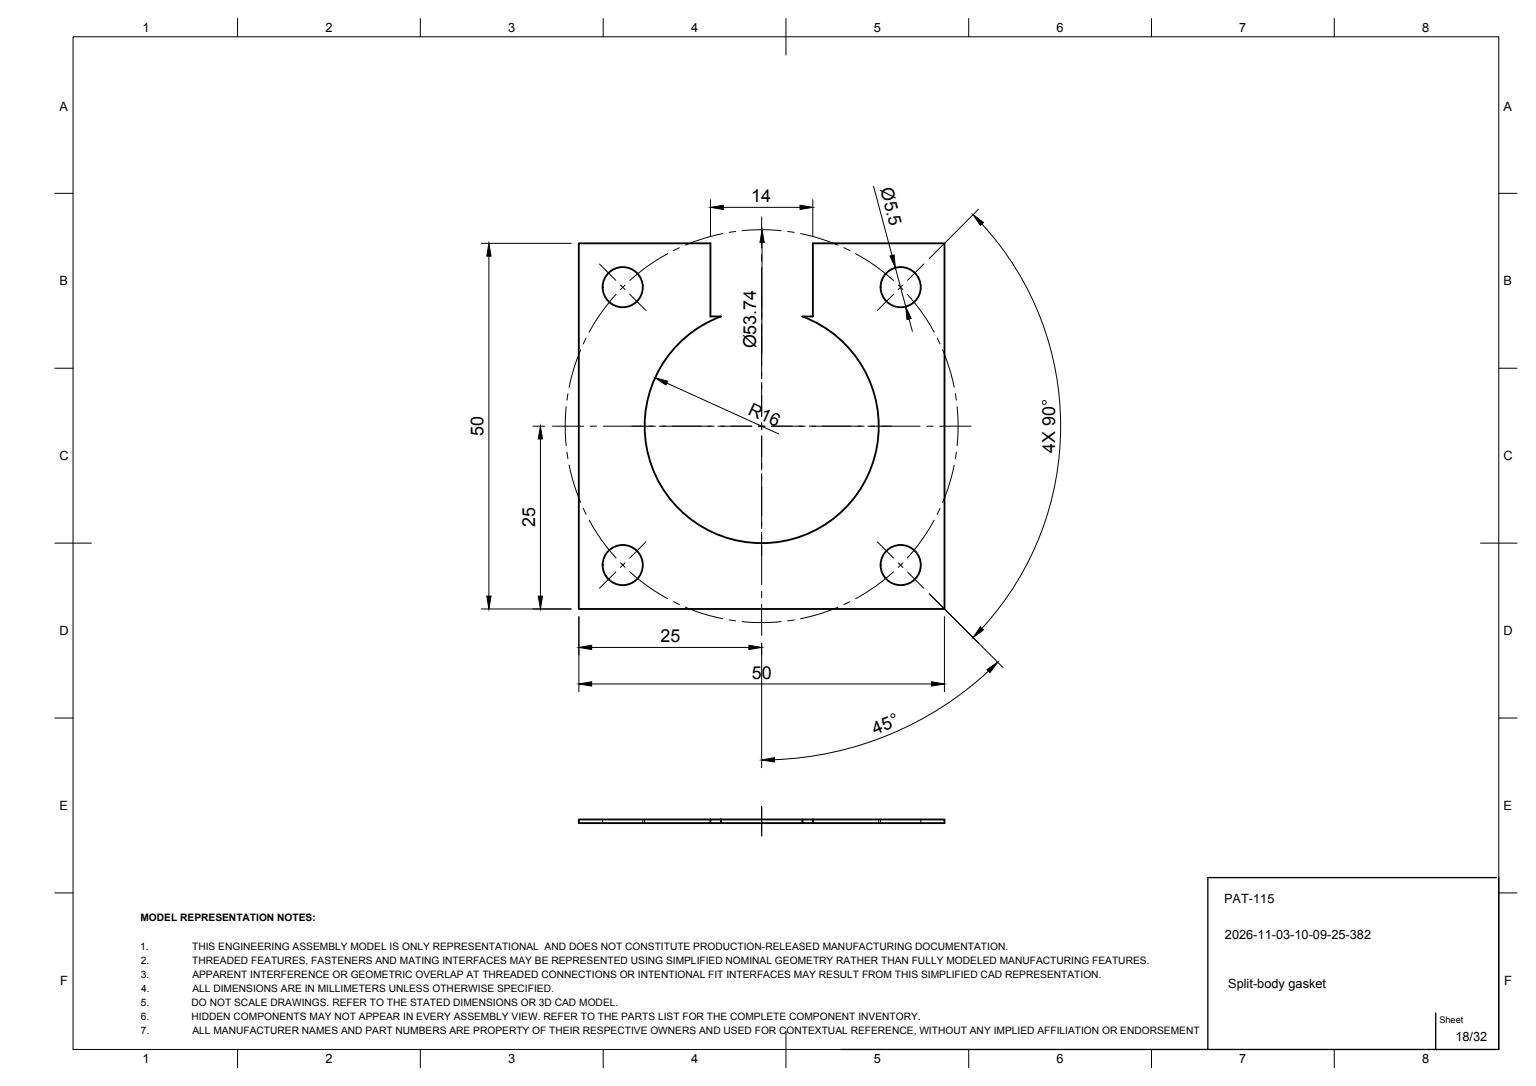
ISO-10303-21;
HEADER;
/* Generated by software containing ST-Developer
 * from STEP Tools, Inc. (www.steptools.com) 
 */

FILE_DESCRIPTION(
/* description */ ('Union bypass pipe loop'),
/* implementation_level */ '2;1');

FILE_NAME(
/* name */ 'Split-body gasket.step',
/* time_stamp */ '2026-10-27T21:00:29-07:00',
/* author */ (''),
/* organization */ (''),
/* preprocessor_version */ 'ST-DEVELOPER v20.2',
/* originating_system */ 'Autodesk Translation Framework v15.17.0.0',
/* authorisation */ '');

FILE_SCHEMA (('AUTOMOTIVE_DESIGN { 1 0 10303 214 3 1 1 }'));
ENDSEC;

DATA;
#10=MECHANICAL_DESIGN_GEOMETRIC_PRESENTATION_REPRESENTATION('',(#447),#10095);
#383=SHAPE_REPRESENTATION_RELATIONSHIP('SRR','None',#10252,#415);
#415=ADVANCED_BREP_SHAPE_REPRESENTATION('',(#479),#10064);
#447=STYLED_ITEM('',(#10479),#479);
#479=MANIFOLD_SOLID_BREP('Body1',#5518);
#539=FACE_BOUND('',#1246,.T.);
#540=FACE_BOUND('',#1247,.T.);
#541=FACE_BOUND('',#1248,.T.);
#542=FACE_BOUND('',#1249,.T.);
#543=FACE_BOUND('',#1257,.T.);
#544=FACE_BOUND('',#1258,.T.);
#545=FACE_BOUND('',#1259,.T.);
#546=FACE_BOUND('',#1260,.T.);
#657=PLANE('',#6007);
#658=PLANE('',#6008);
#659=PLANE('',#6009);
#660=PLANE('',#6010);
#661=PLANE('',#6011);
#662=PLANE('',#6013);
#663=PLANE('',#6014);
#664=PLANE('',#6017);
#665=PLANE('',#6018);
#666=PLANE('',#6019);
#667=PLANE('',#6020);
#877=FACE_OUTER_BOUND('',#1237,.T.);
#878=FACE_OUTER_BOUND('',#1238,.T.);
#879=FACE_OUTER_BOUND('',#1239,.T.);
#880=FACE_OUTER_BOUND('',#1240,.T.);
#881=FACE_OUTER_BOUND('',#1241,.T.);
#882=FACE_OUTER_BOUND('',#1242,.T.);
#883=FACE_OUTER_BOUND('',#1243,.T.);
#884=FACE_OUTER_BOUND('',#1244,.T.);
#885=FACE_OUTER_BOUND('',#1245,.T.);
#886=FACE_OUTER_BOUND('',#1250,.T.);
#887=FACE_OUTER_BOUND('',#1251,.T.);
#888=FACE_OUTER_BOUND('',#1252,.T.);
#889=FACE_OUTER_BOUND('',#1253,.T.);
#890=FACE_OUTER_BOUND('',#1254,.T.);
#891=FACE_OUTER_BOUND('',#1255,.T.);
#892=FACE_OUTER_BOUND('',#1256,.T.);
#1237=EDGE_LOOP('',(#3922,#3923,#3924,#3925));
#1238=EDGE_LOOP('',(#3926,#3927,#3928,#3929));
#1239=EDGE_LOOP('',(#3930,#3931,#3932,#3933));
#1240=EDGE_LOOP('',(#3934,#3935,#3936,#3937));
#1241=EDGE_LOOP('',(#3938,#3939,#3940,#3941));
#1242=EDGE_LOOP('',(#3942,#3943,#3944,#3945));
#1243=EDGE_LOOP('',(#3946,#3947,#3948,#3949));
#1244=EDGE_LOOP('',(#3950,#3951,#3952,#3953));
#1245=EDGE_LOOP('',(#3954,#3955,#3956,#3957,#3958,#3959,#3960,#3961,#3962,
#3963));
#1246=EDGE_LOOP('',(#3964));
#1247=EDGE_LOOP('',(#3965));
#1248=EDGE_LOOP('',(#3966));
#1249=EDGE_LOOP('',(#3967));
#1250=EDGE_LOOP('',(#3968,#3969,#3970,#3971));
#1251=EDGE_LOOP('',(#3972,#3973,#3974,#3975));
#1252=EDGE_LOOP('',(#3976,#3977,#3978,#3979));
#1253=EDGE_LOOP('',(#3980,#3981,#3982,#3983));
#1254=EDGE_LOOP('',(#3984,#3985,#3986,#3987));
#1255=EDGE_LOOP('',(#3988,#3989,#3990,#3991));
#1256=EDGE_LOOP('',(#3992,#3993,#3994,#3995,#3996,#3997,#3998,#3999,#4000,
#4001));
#1257=EDGE_LOOP('',(#4002));
#1258=EDGE_LOOP('',(#4003));
#1259=EDGE_LOOP('',(#4004));
#1260=EDGE_LOOP('',(#4005));
#1673=LINE('',#8629,#2049);
#1674=LINE('',#8635,#2050);
#1675=LINE('',#8641,#2051);
#1676=LINE('',#8647,#2052);
#1677=LINE('',#8652,#2053);
#1678=LINE('',#8654,#2054);
#1679=LINE('',#8656,#2055);
#1680=LINE('',#8657,#2056);
#1681=LINE('',#8661,#2057);
#1682=LINE('',#8663,#2058);
#1683=LINE('',#8665,#2059);
#1684=LINE('',#8666,#2060);
#1685=LINE('',#8669,#2061);
#1686=LINE('',#8671,#2062);
#1687=LINE('',#8672,#2063);
#1688=LINE('',#8675,#2064);
#1689=LINE('',#8677,#2065);
#1690=LINE('',#8678,#2066);
#1691=LINE('',#8682,#2067);
#1692=LINE('',#8684,#2068);
#1693=LINE('',#8686,#2069);
#1694=LINE('',#8688,#2070);
#1695=LINE('',#8689,#2071);
#1696=LINE('',#8692,#2072);
#1697=LINE('',#8693,#2073);
#1698=LINE('',#8696,#2074);
#1699=LINE('',#8697,#2075);
#1700=LINE('',#8702,#2076);
#1701=LINE('',#8703,#2077);
#1702=LINE('',#8706,#2078);
#1703=LINE('',#8707,#2079);
#1704=LINE('',#8709,#2080);
#2049=VECTOR('',#6853,0.275);
#2050=VECTOR('',#6860,0.275);
#2051=VECTOR('',#6867,0.275);
#2052=VECTOR('',#6874,0.275);
#2053=VECTOR('',#6879,1.);
#2054=VECTOR('',#6880,1.);
#2055=VECTOR('',#6881,1.);
#2056=VECTOR('',#6882,1.);
#2057=VECTOR('',#6885,1.);
#2058=VECTOR('',#6886,1.);
#2059=VECTOR('',#6887,1.);
#2060=VECTOR('',#6888,1.);
#2061=VECTOR('',#6891,1.);
#2062=VECTOR('',#6892,1.);
#2063=VECTOR('',#6893,1.);
#2064=VECTOR('',#6896,1.);
#2065=VECTOR('',#6897,1.);
#2066=VECTOR('',#6898,1.);
#2067=VECTOR('',#6903,1.);
#2068=VECTOR('',#6904,1.);
#2069=VECTOR('',#6905,1.);
#2070=VECTOR('',#6906,1.);
#2071=VECTOR('',#6907,1.);
#2072=VECTOR('',#6910,1.);
#2073=VECTOR('',#6911,1.);
#2074=VECTOR('',#6914,1.);
#2075=VECTOR('',#6915,1.);
#2076=VECTOR('',#6922,1.);
#2077=VECTOR('',#6923,1.);
#2078=VECTOR('',#6926,1.);
#2079=VECTOR('',#6927,1.);
#2080=VECTOR('',#6930,1.);
#2417=CIRCLE('',#5996,0.275);
#2418=CIRCLE('',#5997,0.275);
#2419=CIRCLE('',#5999,0.275);
#2420=CIRCLE('',#6000,0.275);
#2421=CIRCLE('',#6002,0.275);
#2422=CIRCLE('',#6003,0.275);
#2423=CIRCLE('',#6005,0.275);
#2424=CIRCLE('',#6006,0.275);
#2425=CIRCLE('',#6012,1.6);
#2426=CIRCLE('',#6016,1.6);
#2692=VERTEX_POINT('',#8626);
#2693=VERTEX_POINT('',#8628);
#2694=VERTEX_POINT('',#8632);
#2695=VERTEX_POINT('',#8634);
#2696=VERTEX_POINT('',#8638);
#2697=VERTEX_POINT('',#8640);
#2698=VERTEX_POINT('',#8644);
#2699=VERTEX_POINT('',#8646);
#2700=VERTEX_POINT('',#8650);
#2701=VERTEX_POINT('',#8651);
#2702=VERTEX_POINT('',#8653);
#2703=VERTEX_POINT('',#8655);
#2704=VERTEX_POINT('',#8659);
#2705=VERTEX_POINT('',#8660);
#2706=VERTEX_POINT('',#8662);
#2707=VERTEX_POINT('',#8664);
#2708=VERTEX_POINT('',#8668);
#2709=VERTEX_POINT('',#8670);
#2710=VERTEX_POINT('',#8674);
#2711=VERTEX_POINT('',#8676);
#2712=VERTEX_POINT('',#8681);
#2713=VERTEX_POINT('',#8683);
#2714=VERTEX_POINT('',#8685);
#2715=VERTEX_POINT('',#8687);
#2716=VERTEX_POINT('',#8691);
#2717=VERTEX_POINT('',#8695);
#2718=VERTEX_POINT('',#8701);
#2719=VERTEX_POINT('',#8705);
#3159=EDGE_CURVE('',#2692,#2692,#2417,.T.);
#3160=EDGE_CURVE('',#2692,#2693,#1673,.T.);
#3161=EDGE_CURVE('',#2693,#2693,#2418,.T.);
#3162=EDGE_CURVE('',#2694,#2694,#2419,.T.);
#3163=EDGE_CURVE('',#2694,#2695,#1674,.T.);
#3164=EDGE_CURVE('',#2695,#2695,#2420,.T.);
#3165=EDGE_CURVE('',#2696,#2696,#2421,.T.);
#3166=EDGE_CURVE('',#2696,#2697,#1675,.T.);
#3167=EDGE_CURVE('',#2697,#2697,#2422,.T.);
#3168=EDGE_CURVE('',#2698,#2698,#2423,.T.);
#3169=EDGE_CURVE('',#2698,#2699,#1676,.T.);
#3170=EDGE_CURVE('',#2699,#2699,#2424,.T.);
#3171=EDGE_CURVE('',#2700,#2701,#1677,.T.);
#3172=EDGE_CURVE('',#2700,#2702,#1678,.T.);
#3173=EDGE_CURVE('',#2703,#2702,#1679,.T.);
#3174=EDGE_CURVE('',#2701,#2703,#1680,.T.);
#3175=EDGE_CURVE('',#2704,#2705,#1681,.T.);
#3176=EDGE_CURVE('',#2704,#2706,#1682,.T.);
#3177=EDGE_CURVE('',#2707,#2706,#1683,.T.);
#3178=EDGE_CURVE('',#2705,#2707,#1684,.T.);
#3179=EDGE_CURVE('',#2708,#2700,#1685,.T.);
#3180=EDGE_CURVE('',#2709,#2708,#1686,.T.);
#3181=EDGE_CURVE('',#2702,#2709,#1687,.T.);
#3182=EDGE_CURVE('',#2710,#2704,#1688,.T.);
#3183=EDGE_CURVE('',#2711,#2710,#1689,.T.);
#3184=EDGE_CURVE('',#2706,#2711,#1690,.T.);
#3185=EDGE_CURVE('',#2709,#2707,#2425,.T.);
#3186=EDGE_CURVE('',#2711,#2712,#1691,.T.);
#3187=EDGE_CURVE('',#2712,#2713,#1692,.T.);
#3188=EDGE_CURVE('',#2713,#2714,#1693,.T.);
#3189=EDGE_CURVE('',#2714,#2715,#1694,.T.);
#3190=EDGE_CURVE('',#2715,#2703,#1695,.T.);
#3191=EDGE_CURVE('',#2716,#2710,#1696,.T.);
#3192=EDGE_CURVE('',#2716,#2712,#1697,.T.);
#3193=EDGE_CURVE('',#2717,#2715,#1698,.T.);
#3194=EDGE_CURVE('',#2701,#2717,#1699,.T.);
#3195=EDGE_CURVE('',#2705,#2708,#2426,.T.);
#3196=EDGE_CURVE('',#2717,#2718,#1700,.T.);
#3197=EDGE_CURVE('',#2718,#2714,#1701,.T.);
#3198=EDGE_CURVE('',#2718,#2719,#1702,.T.);
#3199=EDGE_CURVE('',#2719,#2713,#1703,.T.);
#3200=EDGE_CURVE('',#2719,#2716,#1704,.T.);
#3922=ORIENTED_EDGE('',*,*,#3159,.F.);
#3923=ORIENTED_EDGE('',*,*,#3160,.T.);
#3924=ORIENTED_EDGE('',*,*,#3161,.F.);
#3925=ORIENTED_EDGE('',*,*,#3160,.F.);
#3926=ORIENTED_EDGE('',*,*,#3162,.F.);
#3927=ORIENTED_EDGE('',*,*,#3163,.T.);
#3928=ORIENTED_EDGE('',*,*,#3164,.F.);
#3929=ORIENTED_EDGE('',*,*,#3163,.F.);
#3930=ORIENTED_EDGE('',*,*,#3165,.F.);
#3931=ORIENTED_EDGE('',*,*,#3166,.T.);
#3932=ORIENTED_EDGE('',*,*,#3167,.F.);
#3933=ORIENTED_EDGE('',*,*,#3166,.F.);
#3934=ORIENTED_EDGE('',*,*,#3168,.F.);
#3935=ORIENTED_EDGE('',*,*,#3169,.T.);
#3936=ORIENTED_EDGE('',*,*,#3170,.F.);
#3937=ORIENTED_EDGE('',*,*,#3169,.F.);
#3938=ORIENTED_EDGE('',*,*,#3171,.F.);
#3939=ORIENTED_EDGE('',*,*,#3172,.T.);
#3940=ORIENTED_EDGE('',*,*,#3173,.F.);
#3941=ORIENTED_EDGE('',*,*,#3174,.F.);
#3942=ORIENTED_EDGE('',*,*,#3175,.F.);
#3943=ORIENTED_EDGE('',*,*,#3176,.T.);
#3944=ORIENTED_EDGE('',*,*,#3177,.F.);
#3945=ORIENTED_EDGE('',*,*,#3178,.F.);
#3946=ORIENTED_EDGE('',*,*,#3179,.F.);
#3947=ORIENTED_EDGE('',*,*,#3180,.F.);
#3948=ORIENTED_EDGE('',*,*,#3181,.F.);
#3949=ORIENTED_EDGE('',*,*,#3172,.F.);
#3950=ORIENTED_EDGE('',*,*,#3182,.F.);
#3951=ORIENTED_EDGE('',*,*,#3183,.F.);
#3952=ORIENTED_EDGE('',*,*,#3184,.F.);
#3953=ORIENTED_EDGE('',*,*,#3176,.F.);
#3954=ORIENTED_EDGE('',*,*,#3173,.T.);
#3955=ORIENTED_EDGE('',*,*,#3181,.T.);
#3956=ORIENTED_EDGE('',*,*,#3185,.T.);
#3957=ORIENTED_EDGE('',*,*,#3177,.T.);
#3958=ORIENTED_EDGE('',*,*,#3184,.T.);
#3959=ORIENTED_EDGE('',*,*,#3186,.T.);
#3960=ORIENTED_EDGE('',*,*,#3187,.T.);
#3961=ORIENTED_EDGE('',*,*,#3188,.T.);
#3962=ORIENTED_EDGE('',*,*,#3189,.T.);
#3963=ORIENTED_EDGE('',*,*,#3190,.T.);
#3964=ORIENTED_EDGE('',*,*,#3161,.T.);
#3965=ORIENTED_EDGE('',*,*,#3164,.T.);
#3966=ORIENTED_EDGE('',*,*,#3167,.T.);
#3967=ORIENTED_EDGE('',*,*,#3170,.T.);
#3968=ORIENTED_EDGE('',*,*,#3183,.T.);
#3969=ORIENTED_EDGE('',*,*,#3191,.F.);
#3970=ORIENTED_EDGE('',*,*,#3192,.T.);
#3971=ORIENTED_EDGE('',*,*,#3186,.F.);
#3972=ORIENTED_EDGE('',*,*,#3174,.T.);
#3973=ORIENTED_EDGE('',*,*,#3190,.F.);
#3974=ORIENTED_EDGE('',*,*,#3193,.F.);
#3975=ORIENTED_EDGE('',*,*,#3194,.F.);
#3976=ORIENTED_EDGE('',*,*,#3180,.T.);
#3977=ORIENTED_EDGE('',*,*,#3195,.F.);
#3978=ORIENTED_EDGE('',*,*,#3178,.T.);
#3979=ORIENTED_EDGE('',*,*,#3185,.F.);
#3980=ORIENTED_EDGE('',*,*,#3196,.F.);
#3981=ORIENTED_EDGE('',*,*,#3193,.T.);
#3982=ORIENTED_EDGE('',*,*,#3189,.F.);
#3983=ORIENTED_EDGE('',*,*,#3197,.F.);
#3984=ORIENTED_EDGE('',*,*,#3198,.F.);
#3985=ORIENTED_EDGE('',*,*,#3197,.T.);
#3986=ORIENTED_EDGE('',*,*,#3188,.F.);
#3987=ORIENTED_EDGE('',*,*,#3199,.F.);
#3988=ORIENTED_EDGE('',*,*,#3200,.F.);
#3989=ORIENTED_EDGE('',*,*,#3199,.T.);
#3990=ORIENTED_EDGE('',*,*,#3187,.F.);
#3991=ORIENTED_EDGE('',*,*,#3192,.F.);
#3992=ORIENTED_EDGE('',*,*,#3171,.T.);
#3993=ORIENTED_EDGE('',*,*,#3194,.T.);
#3994=ORIENTED_EDGE('',*,*,#3196,.T.);
#3995=ORIENTED_EDGE('',*,*,#3198,.T.);
#3996=ORIENTED_EDGE('',*,*,#3200,.T.);
#3997=ORIENTED_EDGE('',*,*,#3191,.T.);
#3998=ORIENTED_EDGE('',*,*,#3182,.T.);
#3999=ORIENTED_EDGE('',*,*,#3175,.T.);
#4000=ORIENTED_EDGE('',*,*,#3195,.T.);
#4001=ORIENTED_EDGE('',*,*,#3179,.T.);
#4002=ORIENTED_EDGE('',*,*,#3159,.T.);
#4003=ORIENTED_EDGE('',*,*,#3162,.T.);
#4004=ORIENTED_EDGE('',*,*,#3165,.T.);
#4005=ORIENTED_EDGE('',*,*,#3168,.T.);
#5098=CYLINDRICAL_SURFACE('',#5995,0.275);
#5099=CYLINDRICAL_SURFACE('',#5998,0.275);
#5100=CYLINDRICAL_SURFACE('',#6001,0.275);
#5101=CYLINDRICAL_SURFACE('',#6004,0.275);
#5102=CYLINDRICAL_SURFACE('',#6015,1.6);
#5226=ADVANCED_FACE('',(#877),#5098,.F.);
#5227=ADVANCED_FACE('',(#878),#5099,.F.);
#5228=ADVANCED_FACE('',(#879),#5100,.F.);
#5229=ADVANCED_FACE('',(#880),#5101,.F.);
#5230=ADVANCED_FACE('',(#881),#657,.F.);
#5231=ADVANCED_FACE('',(#882),#658,.F.);
#5232=ADVANCED_FACE('',(#883),#659,.F.);
#5233=ADVANCED_FACE('',(#884),#660,.F.);
#5234=ADVANCED_FACE('',(#885,#539,#540,#541,#542),#661,.T.);
#5235=ADVANCED_FACE('',(#886),#662,.T.);
#5236=ADVANCED_FACE('',(#887),#663,.T.);
#5237=ADVANCED_FACE('',(#888),#5102,.F.);
#5238=ADVANCED_FACE('',(#889),#664,.T.);
#5239=ADVANCED_FACE('',(#890),#665,.T.);
#5240=ADVANCED_FACE('',(#891),#666,.T.);
#5241=ADVANCED_FACE('',(#892,#543,#544,#545,#546),#667,.F.);
#5518=CLOSED_SHELL('',(#5226,#5227,#5228,#5229,#5230,#5231,#5232,#5233,
#5234,#5235,#5236,#5237,#5238,#5239,#5240,#5241));
#5994=AXIS2_PLACEMENT_3D('',#8624,#6847,#6848);
#5995=AXIS2_PLACEMENT_3D('',#8625,#6849,#6850);
#5996=AXIS2_PLACEMENT_3D('',#8627,#6851,#6852);
#5997=AXIS2_PLACEMENT_3D('',#8630,#6854,#6855);
#5998=AXIS2_PLACEMENT_3D('',#8631,#6856,#6857);
#5999=AXIS2_PLACEMENT_3D('',#8633,#6858,#6859);
#6000=AXIS2_PLACEMENT_3D('',#8636,#6861,#6862);
#6001=AXIS2_PLACEMENT_3D('',#8637,#6863,#6864);
#6002=AXIS2_PLACEMENT_3D('',#8639,#6865,#6866);
#6003=AXIS2_PLACEMENT_3D('',#8642,#6868,#6869);
#6004=AXIS2_PLACEMENT_3D('',#8643,#6870,#6871);
#6005=AXIS2_PLACEMENT_3D('',#8645,#6872,#6873);
#6006=AXIS2_PLACEMENT_3D('',#8648,#6875,#6876);
#6007=AXIS2_PLACEMENT_3D('',#8649,#6877,#6878);
#6008=AXIS2_PLACEMENT_3D('',#8658,#6883,#6884);
#6009=AXIS2_PLACEMENT_3D('',#8667,#6889,#6890);
#6010=AXIS2_PLACEMENT_3D('',#8673,#6894,#6895);
#6011=AXIS2_PLACEMENT_3D('',#8679,#6899,#6900);
#6012=AXIS2_PLACEMENT_3D('',#8680,#6901,#6902);
#6013=AXIS2_PLACEMENT_3D('',#8690,#6908,#6909);
#6014=AXIS2_PLACEMENT_3D('',#8694,#6912,#6913);
#6015=AXIS2_PLACEMENT_3D('',#8698,#6916,#6917);
#6016=AXIS2_PLACEMENT_3D('',#8699,#6918,#6919);
#6017=AXIS2_PLACEMENT_3D('',#8700,#6920,#6921);
#6018=AXIS2_PLACEMENT_3D('',#8704,#6924,#6925);
#6019=AXIS2_PLACEMENT_3D('',#8708,#6928,#6929);
#6020=AXIS2_PLACEMENT_3D('',#8710,#6931,#6932);
#6847=DIRECTION('axis',(0.,0.,1.));
#6848=DIRECTION('refdir',(1.,0.,0.));
#6849=DIRECTION('center_axis',(0.,1.,0.));
#6850=DIRECTION('ref_axis',(1.,0.,0.));
#6851=DIRECTION('center_axis',(0.,1.,0.));
#6852=DIRECTION('ref_axis',(1.,0.,0.));
#6853=DIRECTION('',(0.,1.,0.));
#6854=DIRECTION('center_axis',(0.,-1.,0.));
#6855=DIRECTION('ref_axis',(1.,0.,0.));
#6856=DIRECTION('center_axis',(0.,1.,0.));
#6857=DIRECTION('ref_axis',(1.,0.,0.));
#6858=DIRECTION('center_axis',(0.,1.,0.));
#6859=DIRECTION('ref_axis',(1.,0.,0.));
#6860=DIRECTION('',(0.,1.,0.));
#6861=DIRECTION('center_axis',(0.,-1.,0.));
#6862=DIRECTION('ref_axis',(1.,0.,0.));
#6863=DIRECTION('center_axis',(0.,1.,0.));
#6864=DIRECTION('ref_axis',(1.,0.,0.));
#6865=DIRECTION('center_axis',(0.,1.,0.));
#6866=DIRECTION('ref_axis',(1.,0.,0.));
#6867=DIRECTION('',(0.,1.,0.));
#6868=DIRECTION('center_axis',(0.,-1.,0.));
#6869=DIRECTION('ref_axis',(1.,0.,0.));
#6870=DIRECTION('center_axis',(0.,1.,0.));
#6871=DIRECTION('ref_axis',(1.,0.,0.));
#6872=DIRECTION('center_axis',(0.,1.,0.));
#6873=DIRECTION('ref_axis',(1.,0.,0.));
#6874=DIRECTION('',(0.,1.,0.));
#6875=DIRECTION('center_axis',(0.,-1.,0.));
#6876=DIRECTION('ref_axis',(1.,0.,0.));
#6877=DIRECTION('center_axis',(-1.,0.,0.));
#6878=DIRECTION('ref_axis',(0.,0.,1.));
#6879=DIRECTION('',(0.,0.,1.));
#6880=DIRECTION('',(0.,1.,0.));
#6881=DIRECTION('',(0.,0.,-1.));
#6882=DIRECTION('',(0.,1.,0.));
#6883=DIRECTION('center_axis',(0.,0.,-1.));
#6884=DIRECTION('ref_axis',(-1.,0.,0.));
#6885=DIRECTION('',(-1.,0.,0.));
#6886=DIRECTION('',(0.,1.,0.));
#6887=DIRECTION('',(1.,0.,0.));
#6888=DIRECTION('',(0.,1.,0.));
#6889=DIRECTION('center_axis',(0.,0.,-1.));
#6890=DIRECTION('ref_axis',(-1.,0.,0.));
#6891=DIRECTION('',(-1.,0.,0.));
#6892=DIRECTION('',(0.,-1.,0.));
#6893=DIRECTION('',(1.,0.,0.));
#6894=DIRECTION('center_axis',(1.,0.,0.));
#6895=DIRECTION('ref_axis',(0.,0.,-1.));
#6896=DIRECTION('',(0.,0.,-1.));
#6897=DIRECTION('',(0.,-1.,0.));
#6898=DIRECTION('',(0.,0.,1.));
#6899=DIRECTION('center_axis',(0.,1.,0.));
#6900=DIRECTION('ref_axis',(0.,0.,1.));
#6901=DIRECTION('center_axis',(0.,-1.,0.));
#6902=DIRECTION('ref_axis',(1.,0.,0.));
#6903=DIRECTION('',(1.,0.,0.));
#6904=DIRECTION('',(0.,0.,-1.));
#6905=DIRECTION('',(-1.,0.,0.));
#6906=DIRECTION('',(0.,0.,1.));
#6907=DIRECTION('',(1.,0.,0.));
#6908=DIRECTION('center_axis',(0.,0.,1.));
#6909=DIRECTION('ref_axis',(1.,0.,0.));
#6910=DIRECTION('',(-1.,0.,0.));
#6911=DIRECTION('',(0.,1.,0.));
#6912=DIRECTION('center_axis',(0.,0.,1.));
#6913=DIRECTION('ref_axis',(1.,0.,0.));
#6914=DIRECTION('',(0.,1.,0.));
#6915=DIRECTION('',(-1.,0.,0.));
#6916=DIRECTION('center_axis',(0.,1.,0.));
#6917=DIRECTION('ref_axis',(-1.83697019872103E-16,0.,-1.));
#6918=DIRECTION('center_axis',(0.,1.,0.));
#6919=DIRECTION('ref_axis',(1.,0.,0.));
#6920=DIRECTION('center_axis',(-1.,0.,0.));
#6921=DIRECTION('ref_axis',(0.,0.,1.));
#6922=DIRECTION('',(0.,0.,-1.));
#6923=DIRECTION('',(0.,1.,0.));
#6924=DIRECTION('center_axis',(0.,0.,-1.));
#6925=DIRECTION('ref_axis',(-1.,0.,0.));
#6926=DIRECTION('',(1.,0.,0.));
#6927=DIRECTION('',(0.,1.,0.));
#6928=DIRECTION('center_axis',(1.,0.,0.));
#6929=DIRECTION('ref_axis',(0.,0.,-1.));
#6930=DIRECTION('',(0.,0.,1.));
#6931=DIRECTION('center_axis',(0.,1.,0.));
#6932=DIRECTION('ref_axis',(1.,0.,0.));
#8624=CARTESIAN_POINT('',(0.,0.,0.));
#8625=CARTESIAN_POINT('Origin',(1.9,-0.1,3.1));
#8626=CARTESIAN_POINT('',(1.625,-0.025,3.1));
#8627=CARTESIAN_POINT('Origin',(1.9,-0.025,3.1));
#8628=CARTESIAN_POINT('',(1.625,0.025,3.1));
#8629=CARTESIAN_POINT('',(1.625,-0.1,3.1));
#8630=CARTESIAN_POINT('Origin',(1.9,0.025,3.1));
#8631=CARTESIAN_POINT('Origin',(-1.9,-0.1,6.9));
#8632=CARTESIAN_POINT('',(-2.175,-0.025,6.9));
#8633=CARTESIAN_POINT('Origin',(-1.9,-0.025,6.9));
#8634=CARTESIAN_POINT('',(-2.175,0.025,6.9));
#8635=CARTESIAN_POINT('',(-2.175,-0.1,6.9));
#8636=CARTESIAN_POINT('Origin',(-1.9,0.025,6.9));
#8637=CARTESIAN_POINT('Origin',(-1.9,-0.1,3.1));
#8638=CARTESIAN_POINT('',(-2.175,-0.025,3.1));
#8639=CARTESIAN_POINT('Origin',(-1.9,-0.025,3.1));
#8640=CARTESIAN_POINT('',(-2.175,0.025,3.1));
#8641=CARTESIAN_POINT('',(-2.175,-0.1,3.1));
#8642=CARTESIAN_POINT('Origin',(-1.9,0.025,3.1));
#8643=CARTESIAN_POINT('Origin',(1.9,-0.1,6.9));
#8644=CARTESIAN_POINT('',(1.625,-0.025,6.9));
#8645=CARTESIAN_POINT('Origin',(1.9,-0.025,6.9));
#8646=CARTESIAN_POINT('',(1.625,0.025,6.9));
#8647=CARTESIAN_POINT('',(1.625,-0.1,6.9));
#8648=CARTESIAN_POINT('Origin',(1.9,0.025,6.9));
#8649=CARTESIAN_POINT('Origin',(-0.7,-0.1,6.5));
#8650=CARTESIAN_POINT('',(-0.7,-0.025,6.5));
#8651=CARTESIAN_POINT('',(-0.7,-0.025,7.5));
#8652=CARTESIAN_POINT('',(-0.7,-0.025,5.75));
#8653=CARTESIAN_POINT('',(-0.7,0.025,6.5));
#8654=CARTESIAN_POINT('',(-0.7,-0.1,6.5));
#8655=CARTESIAN_POINT('',(-0.7,0.025,7.5));
#8656=CARTESIAN_POINT('',(-0.7,0.025,5.75));
#8657=CARTESIAN_POINT('',(-0.7,-0.0625,7.5));
#8658=CARTESIAN_POINT('Origin',(0.7,-0.1,6.5));
#8659=CARTESIAN_POINT('',(0.7,-0.025,6.5));
#8660=CARTESIAN_POINT('',(0.556776436283003,-0.025,6.5));
#8661=CARTESIAN_POINT('',(0.35,-0.025,6.5));
#8662=CARTESIAN_POINT('',(0.7,0.025,6.5));
#8663=CARTESIAN_POINT('',(0.7,-0.1,6.5));
#8664=CARTESIAN_POINT('',(0.556776436283003,0.025,6.5));
#8665=CARTESIAN_POINT('',(0.35,0.025,6.5));
#8666=CARTESIAN_POINT('',(0.556776436283003,-0.1,6.5));
#8667=CARTESIAN_POINT('Origin',(0.7,-0.1,6.5));
#8668=CARTESIAN_POINT('',(-0.556776436283003,-0.025,6.5));
#8669=CARTESIAN_POINT('',(0.35,-0.025,6.5));
#8670=CARTESIAN_POINT('',(-0.556776436283003,0.025,6.5));
#8671=CARTESIAN_POINT('',(-0.556776436283003,-0.1,6.5));
#8672=CARTESIAN_POINT('',(0.35,0.025,6.5));
#8673=CARTESIAN_POINT('Origin',(0.7,-0.1,7.6));
#8674=CARTESIAN_POINT('',(0.7,-0.025,7.5));
#8675=CARTESIAN_POINT('',(0.7,-0.025,6.3));
#8676=CARTESIAN_POINT('',(0.7,0.025,7.5));
#8677=CARTESIAN_POINT('',(0.7,-0.0625,7.5));
#8678=CARTESIAN_POINT('',(0.7,0.025,6.3));
#8679=CARTESIAN_POINT('Origin',(0.,0.025,5.));
#8680=CARTESIAN_POINT('Origin',(0.,0.025,5.));
#8681=CARTESIAN_POINT('',(2.5,0.025,7.5));
#8682=CARTESIAN_POINT('',(2.5,0.025,7.5));
#8683=CARTESIAN_POINT('',(2.5,0.025,2.5));
#8684=CARTESIAN_POINT('',(2.5,0.025,2.5));
#8685=CARTESIAN_POINT('',(-2.5,0.025,2.5));
#8686=CARTESIAN_POINT('',(-2.5,0.025,2.5));
#8687=CARTESIAN_POINT('',(-2.5,0.025,7.5));
#8688=CARTESIAN_POINT('',(-2.5,0.025,7.5));
#8689=CARTESIAN_POINT('',(2.5,0.025,7.5));
#8690=CARTESIAN_POINT('Origin',(-2.5,-0.025,7.5));
#8691=CARTESIAN_POINT('',(2.5,-0.025,7.5));
#8692=CARTESIAN_POINT('',(2.5,-0.025,7.5));
#8693=CARTESIAN_POINT('',(2.5,-0.025,7.5));
#8694=CARTESIAN_POINT('Origin',(-2.5,-0.025,7.5));
#8695=CARTESIAN_POINT('',(-2.5,-0.025,7.5));
#8696=CARTESIAN_POINT('',(-2.5,-0.025,7.5));
#8697=CARTESIAN_POINT('',(2.5,-0.025,7.5));
#8698=CARTESIAN_POINT('Origin',(0.,-0.1,5.));
#8699=CARTESIAN_POINT('Origin',(0.,-0.025,5.));
#8700=CARTESIAN_POINT('Origin',(-2.5,-0.025,2.5));
#8701=CARTESIAN_POINT('',(-2.5,-0.025,2.5));
#8702=CARTESIAN_POINT('',(-2.5,-0.025,7.5));
#8703=CARTESIAN_POINT('',(-2.5,-0.025,2.5));
#8704=CARTESIAN_POINT('Origin',(2.5,-0.025,2.5));
#8705=CARTESIAN_POINT('',(2.5,-0.025,2.5));
#8706=CARTESIAN_POINT('',(-2.5,-0.025,2.5));
#8707=CARTESIAN_POINT('',(2.5,-0.025,2.5));
#8708=CARTESIAN_POINT('Origin',(2.5,-0.025,7.5));
#8709=CARTESIAN_POINT('',(2.5,-0.025,2.5));
#8710=CARTESIAN_POINT('Origin',(0.,-0.025,5.));
#10027=UNCERTAINTY_MEASURE_WITH_UNIT(LENGTH_MEASURE(0.001),#10096,
'DISTANCE_ACCURACY_VALUE',
'Maximum model space distance between geometric entities at asserted c
onnectivities');
#10058=UNCERTAINTY_MEASURE_WITH_UNIT(LENGTH_MEASURE(0.001),#10096,
'DISTANCE_ACCURACY_VALUE',
'Maximum model space distance between geometric entities at asserted c
onnectivities');
#10064=(
GEOMETRIC_REPRESENTATION_CONTEXT(3)
GLOBAL_UNCERTAINTY_ASSIGNED_CONTEXT((#10027))
GLOBAL_UNIT_ASSIGNED_CONTEXT((#10096,#10098,#10099))
REPRESENTATION_CONTEXT('','3D')
);
#10095=(
GEOMETRIC_REPRESENTATION_CONTEXT(3)
GLOBAL_UNCERTAINTY_ASSIGNED_CONTEXT((#10058))
GLOBAL_UNIT_ASSIGNED_CONTEXT((#10096,#10098,#10099))
REPRESENTATION_CONTEXT('','3D')
);
#10096=(
LENGTH_UNIT()
NAMED_UNIT(*)
SI_UNIT(.CENTI.,.METRE.)
);
#10098=(
NAMED_UNIT(*)
PLANE_ANGLE_UNIT()
SI_UNIT($,.RADIAN.)
);
#10099=(
NAMED_UNIT(*)
SI_UNIT($,.STERADIAN.)
SOLID_ANGLE_UNIT()
);
#10105=SHAPE_DEFINITION_REPRESENTATION(#10141,#10252);
#10141=PRODUCT_DEFINITION_SHAPE('',$,#10289);
#10252=SHAPE_REPRESENTATION('',(#5994),#10064);
#10283=PRODUCT_DEFINITION_CONTEXT('part definition',#10393,'design');
#10289=PRODUCT_DEFINITION('Split-body gasket','Split-body gasket',#10325,
#10283);
#10325=PRODUCT_DEFINITION_FORMATION('',$,#10400);
#10393=APPLICATION_CONTEXT(
'Core Data for Automotive Mechanical Design Process');
#10394=PRODUCT_CONTEXT('part definition',#10393,'mechanical');
#10400=PRODUCT('Split-body gasket','Split-body gasket',
'Split-body gasket',(#10394));
#10473=COLOUR_RGB('Dark Blue',0.08,0.2,0.34);
#10474=FILL_AREA_STYLE_COLOUR('',#10473);
#10475=FILL_AREA_STYLE('',(#10474));
#10476=SURFACE_STYLE_FILL_AREA(#10475);
#10477=SURFACE_SIDE_STYLE('',(#10476));
#10478=SURFACE_STYLE_USAGE(.BOTH.,#10477);
#10479=PRESENTATION_STYLE_ASSIGNMENT((#10478));
ENDSEC;
END-ISO-10303-21;
